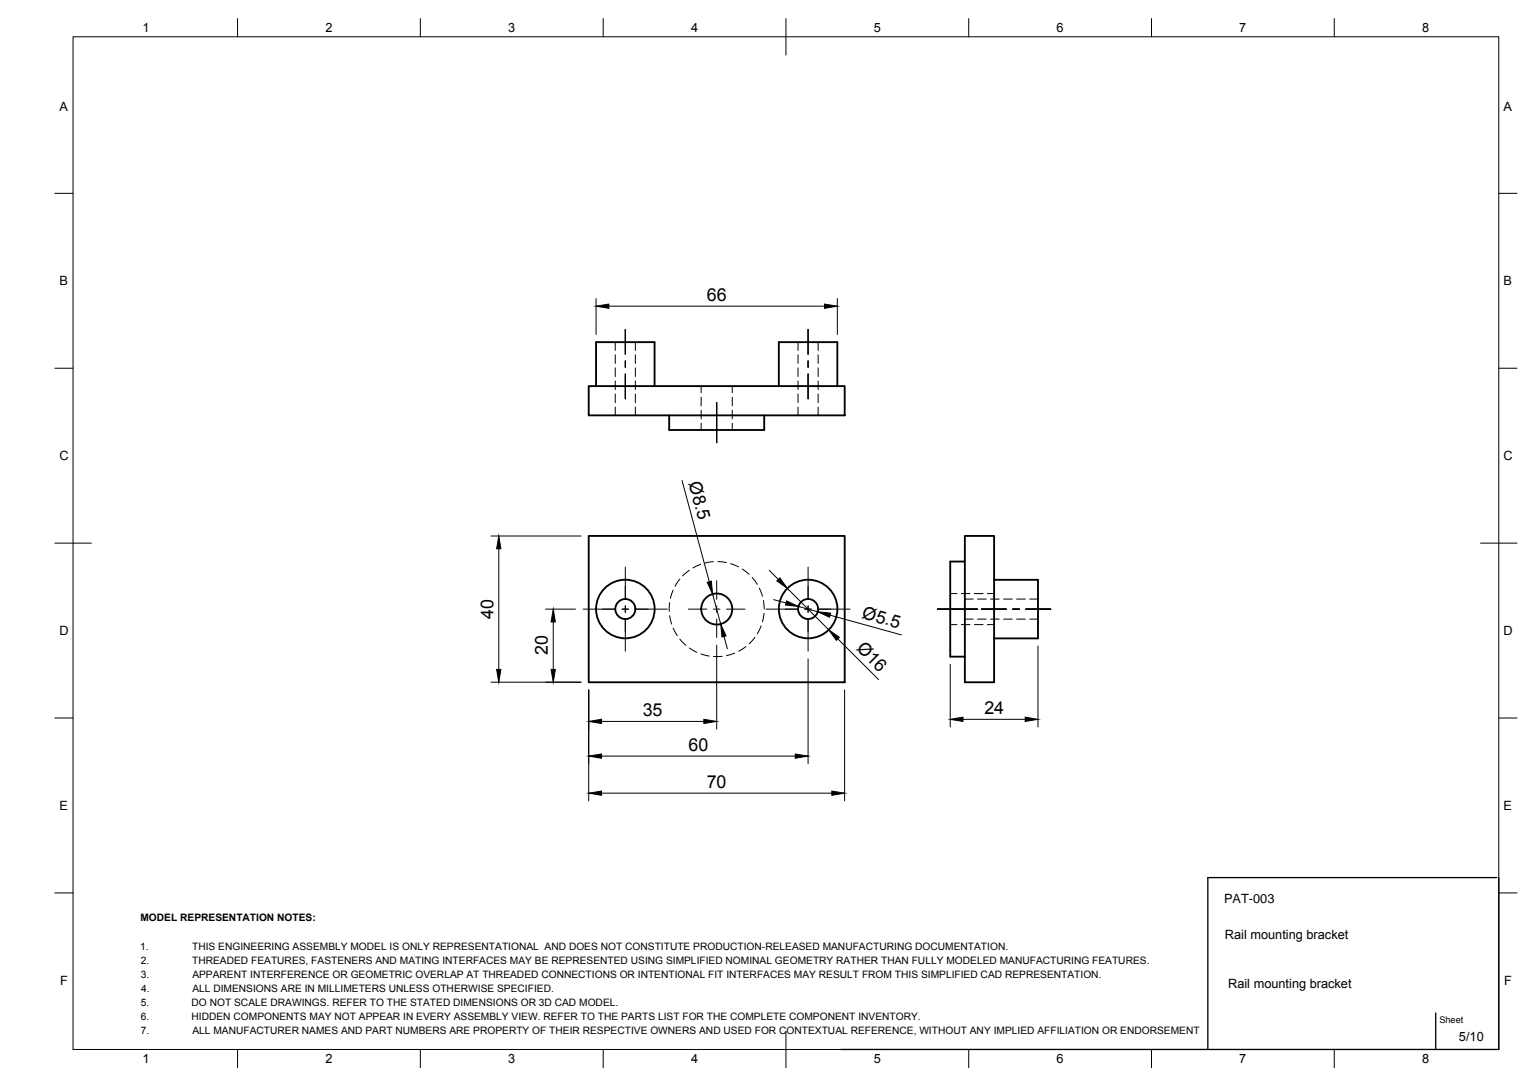
ISO-10303-21;
HEADER;
/* Generated by software containing ST-Developer
 * from STEP Tools, Inc. (www.steptools.com) 
 */

FILE_DESCRIPTION(
/* description */ ('PAT-003'),
/* implementation_level */ '2;1');

FILE_NAME(
/* name */ 'Rail mounting bracket.step',
/* time_stamp */ '2026-10-29T15:45:40-07:00',
/* author */ (''),
/* organization */ (''),
/* preprocessor_version */ 'ST-DEVELOPER v20.2',
/* originating_system */ 'Autodesk Translation Framework v15.17.0.0',
/* authorisation */ '');

FILE_SCHEMA (('AUTOMOTIVE_DESIGN { 1 0 10303 214 3 1 1 }'));
ENDSEC;

DATA;
#10=MECHANICAL_DESIGN_GEOMETRIC_PRESENTATION_REPRESENTATION('',(#147),#5761);
#123=SHAPE_REPRESENTATION_RELATIONSHIP('SRR','None',#5817,#135);
#135=ADVANCED_BREP_SHAPE_REPRESENTATION('',(#159),#5748);
#147=STYLED_ITEM('',(#5928),#159);
#159=MANIFOLD_SOLID_BREP('Body1',#3321);
#169=FACE_BOUND('',#530,.T.);
#170=FACE_BOUND('',#533,.T.);
#171=FACE_BOUND('',#539,.T.);
#172=FACE_BOUND('',#545,.T.);
#173=FACE_BOUND('',#546,.T.);
#174=FACE_BOUND('',#547,.T.);
#175=FACE_BOUND('',#549,.T.);
#176=FACE_BOUND('',#550,.T.);
#177=FACE_BOUND('',#551,.T.);
#206=PLANE('',#3474);
#207=PLANE('',#3479);
#208=PLANE('',#3491);
#209=PLANE('',#3492);
#210=PLANE('',#3493);
#211=PLANE('',#3494);
#212=PLANE('',#3495);
#213=PLANE('',#3496);
#214=PLANE('',#3497);
#341=FACE_OUTER_BOUND('',#528,.T.);
#342=FACE_OUTER_BOUND('',#529,.T.);
#343=FACE_OUTER_BOUND('',#531,.T.);
#344=FACE_OUTER_BOUND('',#532,.T.);
#345=FACE_OUTER_BOUND('',#534,.T.);
#346=FACE_OUTER_BOUND('',#535,.T.);
#347=FACE_OUTER_BOUND('',#536,.T.);
#348=FACE_OUTER_BOUND('',#537,.T.);
#349=FACE_OUTER_BOUND('',#538,.T.);
#350=FACE_OUTER_BOUND('',#540,.T.);
#351=FACE_OUTER_BOUND('',#541,.T.);
#352=FACE_OUTER_BOUND('',#542,.T.);
#353=FACE_OUTER_BOUND('',#543,.T.);
#354=FACE_OUTER_BOUND('',#544,.T.);
#355=FACE_OUTER_BOUND('',#548,.T.);
#528=EDGE_LOOP('',(#2218,#2219,#2220,#2221));
#529=EDGE_LOOP('',(#2222));
#530=EDGE_LOOP('',(#2223));
#531=EDGE_LOOP('',(#2224,#2225,#2226,#2227));
#532=EDGE_LOOP('',(#2228));
#533=EDGE_LOOP('',(#2229));
#534=EDGE_LOOP('',(#2230,#2231,#2232,#2233));
#535=EDGE_LOOP('',(#2234,#2235,#2236,#2237));
#536=EDGE_LOOP('',(#2238,#2239,#2240,#2241));
#537=EDGE_LOOP('',(#2242,#2243,#2244,#2245));
#538=EDGE_LOOP('',(#2246));
#539=EDGE_LOOP('',(#2247));
#540=EDGE_LOOP('',(#2248,#2249,#2250,#2251));
#541=EDGE_LOOP('',(#2252,#2253,#2254,#2255));
#542=EDGE_LOOP('',(#2256,#2257,#2258,#2259));
#543=EDGE_LOOP('',(#2260,#2261,#2262,#2263));
#544=EDGE_LOOP('',(#2264,#2265,#2266,#2267));
#545=EDGE_LOOP('',(#2268));
#546=EDGE_LOOP('',(#2269));
#547=EDGE_LOOP('',(#2270));
#548=EDGE_LOOP('',(#2271,#2272,#2273,#2274));
#549=EDGE_LOOP('',(#2275));
#550=EDGE_LOOP('',(#2276));
#551=EDGE_LOOP('',(#2277));
#752=LINE('',#4754,#1074);
#753=LINE('',#4763,#1075);
#754=LINE('',#4770,#1076);
#755=LINE('',#4774,#1077);
#756=LINE('',#4780,#1078);
#757=LINE('',#4786,#1079);
#758=LINE('',#4792,#1080);
#759=LINE('',#4794,#1081);
#760=LINE('',#4796,#1082);
#761=LINE('',#4797,#1083);
#762=LINE('',#4800,#1084);
#763=LINE('',#4802,#1085);
#764=LINE('',#4803,#1086);
#765=LINE('',#4806,#1087);
#766=LINE('',#4808,#1088);
#767=LINE('',#4809,#1089);
#768=LINE('',#4811,#1090);
#769=LINE('',#4812,#1091);
#1074=VECTOR('',#3797,0.800000000000001);
#1075=VECTOR('',#3808,0.8);
#1076=VECTOR('',#3817,0.275);
#1077=VECTOR('',#3822,0.275);
#1078=VECTOR('',#3829,0.425);
#1079=VECTOR('',#3836,1.3);
#1080=VECTOR('',#3843,1.);
#1081=VECTOR('',#3844,1.);
#1082=VECTOR('',#3845,1.);
#1083=VECTOR('',#3846,1.);
#1084=VECTOR('',#3849,1.);
#1085=VECTOR('',#3850,1.);
#1086=VECTOR('',#3851,1.);
#1087=VECTOR('',#3854,1.);
#1088=VECTOR('',#3855,1.);
#1089=VECTOR('',#3856,1.);
#1090=VECTOR('',#3859,1.);
#1091=VECTOR('',#3860,1.);
#1396=CIRCLE('',#3472,0.800000000000001);
#1397=CIRCLE('',#3473,0.800000000000001);
#1398=CIRCLE('',#3475,0.275);
#1399=CIRCLE('',#3477,0.8);
#1400=CIRCLE('',#3478,0.8);
#1401=CIRCLE('',#3480,0.275);
#1402=CIRCLE('',#3482,0.275);
#1403=CIRCLE('',#3484,0.275);
#1404=CIRCLE('',#3486,0.425);
#1405=CIRCLE('',#3487,0.425);
#1406=CIRCLE('',#3489,1.3);
#1407=CIRCLE('',#3490,1.3);
#1492=VERTEX_POINT('',#4751);
#1493=VERTEX_POINT('',#4753);
#1494=VERTEX_POINT('',#4757);
#1495=VERTEX_POINT('',#4760);
#1496=VERTEX_POINT('',#4762);
#1497=VERTEX_POINT('',#4766);
#1498=VERTEX_POINT('',#4769);
#1499=VERTEX_POINT('',#4773);
#1500=VERTEX_POINT('',#4777);
#1501=VERTEX_POINT('',#4779);
#1502=VERTEX_POINT('',#4783);
#1503=VERTEX_POINT('',#4785);
#1504=VERTEX_POINT('',#4790);
#1505=VERTEX_POINT('',#4791);
#1506=VERTEX_POINT('',#4793);
#1507=VERTEX_POINT('',#4795);
#1508=VERTEX_POINT('',#4799);
#1509=VERTEX_POINT('',#4801);
#1510=VERTEX_POINT('',#4805);
#1511=VERTEX_POINT('',#4807);
#1780=EDGE_CURVE('',#1492,#1492,#1396,.T.);
#1781=EDGE_CURVE('',#1492,#1493,#752,.T.);
#1782=EDGE_CURVE('',#1493,#1493,#1397,.T.);
#1783=EDGE_CURVE('',#1494,#1494,#1398,.T.);
#1784=EDGE_CURVE('',#1495,#1495,#1399,.T.);
#1785=EDGE_CURVE('',#1495,#1496,#753,.T.);
#1786=EDGE_CURVE('',#1496,#1496,#1400,.T.);
#1787=EDGE_CURVE('',#1497,#1497,#1401,.T.);
#1788=EDGE_CURVE('',#1497,#1498,#754,.T.);
#1789=EDGE_CURVE('',#1498,#1498,#1402,.T.);
#1790=EDGE_CURVE('',#1494,#1499,#755,.T.);
#1791=EDGE_CURVE('',#1499,#1499,#1403,.T.);
#1792=EDGE_CURVE('',#1500,#1500,#1404,.T.);
#1793=EDGE_CURVE('',#1500,#1501,#756,.T.);
#1794=EDGE_CURVE('',#1501,#1501,#1405,.T.);
#1795=EDGE_CURVE('',#1502,#1502,#1406,.T.);
#1796=EDGE_CURVE('',#1502,#1503,#757,.T.);
#1797=EDGE_CURVE('',#1503,#1503,#1407,.T.);
#1798=EDGE_CURVE('',#1504,#1505,#758,.T.);
#1799=EDGE_CURVE('',#1505,#1506,#759,.T.);
#1800=EDGE_CURVE('',#1507,#1506,#760,.T.);
#1801=EDGE_CURVE('',#1504,#1507,#761,.T.);
#1802=EDGE_CURVE('',#1508,#1504,#762,.T.);
#1803=EDGE_CURVE('',#1509,#1507,#763,.T.);
#1804=EDGE_CURVE('',#1508,#1509,#764,.T.);
#1805=EDGE_CURVE('',#1510,#1508,#765,.T.);
#1806=EDGE_CURVE('',#1511,#1509,#766,.T.);
#1807=EDGE_CURVE('',#1510,#1511,#767,.T.);
#1808=EDGE_CURVE('',#1505,#1510,#768,.T.);
#1809=EDGE_CURVE('',#1506,#1511,#769,.T.);
#2218=ORIENTED_EDGE('',*,*,#1780,.F.);
#2219=ORIENTED_EDGE('',*,*,#1781,.T.);
#2220=ORIENTED_EDGE('',*,*,#1782,.T.);
#2221=ORIENTED_EDGE('',*,*,#1781,.F.);
#2222=ORIENTED_EDGE('',*,*,#1782,.F.);
#2223=ORIENTED_EDGE('',*,*,#1783,.F.);
#2224=ORIENTED_EDGE('',*,*,#1784,.F.);
#2225=ORIENTED_EDGE('',*,*,#1785,.T.);
#2226=ORIENTED_EDGE('',*,*,#1786,.T.);
#2227=ORIENTED_EDGE('',*,*,#1785,.F.);
#2228=ORIENTED_EDGE('',*,*,#1786,.F.);
#2229=ORIENTED_EDGE('',*,*,#1787,.F.);
#2230=ORIENTED_EDGE('',*,*,#1787,.T.);
#2231=ORIENTED_EDGE('',*,*,#1788,.T.);
#2232=ORIENTED_EDGE('',*,*,#1789,.F.);
#2233=ORIENTED_EDGE('',*,*,#1788,.F.);
#2234=ORIENTED_EDGE('',*,*,#1783,.T.);
#2235=ORIENTED_EDGE('',*,*,#1790,.T.);
#2236=ORIENTED_EDGE('',*,*,#1791,.F.);
#2237=ORIENTED_EDGE('',*,*,#1790,.F.);
#2238=ORIENTED_EDGE('',*,*,#1792,.F.);
#2239=ORIENTED_EDGE('',*,*,#1793,.T.);
#2240=ORIENTED_EDGE('',*,*,#1794,.F.);
#2241=ORIENTED_EDGE('',*,*,#1793,.F.);
#2242=ORIENTED_EDGE('',*,*,#1795,.F.);
#2243=ORIENTED_EDGE('',*,*,#1796,.T.);
#2244=ORIENTED_EDGE('',*,*,#1797,.F.);
#2245=ORIENTED_EDGE('',*,*,#1796,.F.);
#2246=ORIENTED_EDGE('',*,*,#1795,.T.);
#2247=ORIENTED_EDGE('',*,*,#1794,.T.);
#2248=ORIENTED_EDGE('',*,*,#1798,.T.);
#2249=ORIENTED_EDGE('',*,*,#1799,.T.);
#2250=ORIENTED_EDGE('',*,*,#1800,.F.);
#2251=ORIENTED_EDGE('',*,*,#1801,.F.);
#2252=ORIENTED_EDGE('',*,*,#1802,.T.);
#2253=ORIENTED_EDGE('',*,*,#1801,.T.);
#2254=ORIENTED_EDGE('',*,*,#1803,.F.);
#2255=ORIENTED_EDGE('',*,*,#1804,.F.);
#2256=ORIENTED_EDGE('',*,*,#1805,.T.);
#2257=ORIENTED_EDGE('',*,*,#1804,.T.);
#2258=ORIENTED_EDGE('',*,*,#1806,.F.);
#2259=ORIENTED_EDGE('',*,*,#1807,.F.);
#2260=ORIENTED_EDGE('',*,*,#1808,.T.);
#2261=ORIENTED_EDGE('',*,*,#1807,.T.);
#2262=ORIENTED_EDGE('',*,*,#1809,.F.);
#2263=ORIENTED_EDGE('',*,*,#1799,.F.);
#2264=ORIENTED_EDGE('',*,*,#1809,.T.);
#2265=ORIENTED_EDGE('',*,*,#1806,.T.);
#2266=ORIENTED_EDGE('',*,*,#1803,.T.);
#2267=ORIENTED_EDGE('',*,*,#1800,.T.);
#2268=ORIENTED_EDGE('',*,*,#1789,.T.);
#2269=ORIENTED_EDGE('',*,*,#1791,.T.);
#2270=ORIENTED_EDGE('',*,*,#1797,.T.);
#2271=ORIENTED_EDGE('',*,*,#1808,.F.);
#2272=ORIENTED_EDGE('',*,*,#1798,.F.);
#2273=ORIENTED_EDGE('',*,*,#1802,.F.);
#2274=ORIENTED_EDGE('',*,*,#1805,.F.);
#2275=ORIENTED_EDGE('',*,*,#1780,.T.);
#2276=ORIENTED_EDGE('',*,*,#1784,.T.);
#2277=ORIENTED_EDGE('',*,*,#1792,.T.);
#3094=CYLINDRICAL_SURFACE('',#3471,0.800000000000001);
#3095=CYLINDRICAL_SURFACE('',#3476,0.8);
#3096=CYLINDRICAL_SURFACE('',#3481,0.275);
#3097=CYLINDRICAL_SURFACE('',#3483,0.275);
#3098=CYLINDRICAL_SURFACE('',#3485,0.425);
#3099=CYLINDRICAL_SURFACE('',#3488,1.3);
#3134=ADVANCED_FACE('',(#341),#3094,.T.);
#3135=ADVANCED_FACE('',(#342,#169),#206,.F.);
#3136=ADVANCED_FACE('',(#343),#3095,.T.);
#3137=ADVANCED_FACE('',(#344,#170),#207,.F.);
#3138=ADVANCED_FACE('',(#345),#3096,.F.);
#3139=ADVANCED_FACE('',(#346),#3097,.F.);
#3140=ADVANCED_FACE('',(#347),#3098,.F.);
#3141=ADVANCED_FACE('',(#348),#3099,.T.);
#3142=ADVANCED_FACE('',(#349,#171),#208,.T.);
#3143=ADVANCED_FACE('',(#350),#209,.T.);
#3144=ADVANCED_FACE('',(#351),#210,.T.);
#3145=ADVANCED_FACE('',(#352),#211,.T.);
#3146=ADVANCED_FACE('',(#353),#212,.T.);
#3147=ADVANCED_FACE('',(#354,#172,#173,#174),#213,.T.);
#3148=ADVANCED_FACE('',(#355,#175,#176,#177),#214,.F.);
#3321=CLOSED_SHELL('',(#3134,#3135,#3136,#3137,#3138,#3139,#3140,#3141,
#3142,#3143,#3144,#3145,#3146,#3147,#3148));
#3470=AXIS2_PLACEMENT_3D('',#4749,#3791,#3792);
#3471=AXIS2_PLACEMENT_3D('',#4750,#3793,#3794);
#3472=AXIS2_PLACEMENT_3D('',#4752,#3795,#3796);
#3473=AXIS2_PLACEMENT_3D('',#4755,#3798,#3799);
#3474=AXIS2_PLACEMENT_3D('',#4756,#3800,#3801);
#3475=AXIS2_PLACEMENT_3D('',#4758,#3802,#3803);
#3476=AXIS2_PLACEMENT_3D('',#4759,#3804,#3805);
#3477=AXIS2_PLACEMENT_3D('',#4761,#3806,#3807);
#3478=AXIS2_PLACEMENT_3D('',#4764,#3809,#3810);
#3479=AXIS2_PLACEMENT_3D('',#4765,#3811,#3812);
#3480=AXIS2_PLACEMENT_3D('',#4767,#3813,#3814);
#3481=AXIS2_PLACEMENT_3D('',#4768,#3815,#3816);
#3482=AXIS2_PLACEMENT_3D('',#4771,#3818,#3819);
#3483=AXIS2_PLACEMENT_3D('',#4772,#3820,#3821);
#3484=AXIS2_PLACEMENT_3D('',#4775,#3823,#3824);
#3485=AXIS2_PLACEMENT_3D('',#4776,#3825,#3826);
#3486=AXIS2_PLACEMENT_3D('',#4778,#3827,#3828);
#3487=AXIS2_PLACEMENT_3D('',#4781,#3830,#3831);
#3488=AXIS2_PLACEMENT_3D('',#4782,#3832,#3833);
#3489=AXIS2_PLACEMENT_3D('',#4784,#3834,#3835);
#3490=AXIS2_PLACEMENT_3D('',#4787,#3837,#3838);
#3491=AXIS2_PLACEMENT_3D('',#4788,#3839,#3840);
#3492=AXIS2_PLACEMENT_3D('',#4789,#3841,#3842);
#3493=AXIS2_PLACEMENT_3D('',#4798,#3847,#3848);
#3494=AXIS2_PLACEMENT_3D('',#4804,#3852,#3853);
#3495=AXIS2_PLACEMENT_3D('',#4810,#3857,#3858);
#3496=AXIS2_PLACEMENT_3D('',#4813,#3861,#3862);
#3497=AXIS2_PLACEMENT_3D('',#4814,#3863,#3864);
#3791=DIRECTION('axis',(0.,0.,1.));
#3792=DIRECTION('refdir',(1.,0.,0.));
#3793=DIRECTION('center_axis',(0.,0.,1.));
#3794=DIRECTION('ref_axis',(1.,0.,0.));
#3795=DIRECTION('center_axis',(0.,0.,1.));
#3796=DIRECTION('ref_axis',(1.,0.,0.));
#3797=DIRECTION('',(0.,0.,-1.));
#3798=DIRECTION('center_axis',(0.,0.,1.));
#3799=DIRECTION('ref_axis',(1.,0.,0.));
#3800=DIRECTION('center_axis',(0.,0.,1.));
#3801=DIRECTION('ref_axis',(1.,0.,0.));
#3802=DIRECTION('center_axis',(0.,0.,-1.));
#3803=DIRECTION('ref_axis',(1.,0.,0.));
#3804=DIRECTION('center_axis',(0.,0.,1.));
#3805=DIRECTION('ref_axis',(1.,0.,0.));
#3806=DIRECTION('center_axis',(0.,0.,1.));
#3807=DIRECTION('ref_axis',(1.,0.,0.));
#3808=DIRECTION('',(0.,0.,-1.));
#3809=DIRECTION('center_axis',(0.,0.,1.));
#3810=DIRECTION('ref_axis',(1.,0.,0.));
#3811=DIRECTION('center_axis',(0.,0.,1.));
#3812=DIRECTION('ref_axis',(1.,0.,0.));
#3813=DIRECTION('center_axis',(0.,0.,-1.));
#3814=DIRECTION('ref_axis',(1.,0.,0.));
#3815=DIRECTION('center_axis',(0.,0.,1.));
#3816=DIRECTION('ref_axis',(1.,0.,0.));
#3817=DIRECTION('',(0.,0.,1.));
#3818=DIRECTION('center_axis',(0.,0.,-1.));
#3819=DIRECTION('ref_axis',(1.,0.,0.));
#3820=DIRECTION('center_axis',(0.,0.,1.));
#3821=DIRECTION('ref_axis',(1.,0.,0.));
#3822=DIRECTION('',(0.,0.,1.));
#3823=DIRECTION('center_axis',(0.,0.,-1.));
#3824=DIRECTION('ref_axis',(1.,0.,0.));
#3825=DIRECTION('center_axis',(0.,0.,1.));
#3826=DIRECTION('ref_axis',(1.,0.,0.));
#3827=DIRECTION('center_axis',(0.,0.,1.));
#3828=DIRECTION('ref_axis',(1.,0.,0.));
#3829=DIRECTION('',(0.,0.,1.));
#3830=DIRECTION('center_axis',(0.,0.,-1.));
#3831=DIRECTION('ref_axis',(1.,0.,0.));
#3832=DIRECTION('center_axis',(0.,0.,1.));
#3833=DIRECTION('ref_axis',(1.,0.,0.));
#3834=DIRECTION('center_axis',(0.,0.,1.));
#3835=DIRECTION('ref_axis',(1.,0.,0.));
#3836=DIRECTION('',(0.,0.,-1.));
#3837=DIRECTION('center_axis',(0.,0.,-1.));
#3838=DIRECTION('ref_axis',(1.,0.,0.));
#3839=DIRECTION('center_axis',(0.,0.,1.));
#3840=DIRECTION('ref_axis',(1.,0.,0.));
#3841=DIRECTION('center_axis',(0.,1.,0.));
#3842=DIRECTION('ref_axis',(-1.,0.,0.));
#3843=DIRECTION('',(-1.,0.,0.));
#3844=DIRECTION('',(0.,0.,1.));
#3845=DIRECTION('',(-1.,0.,0.));
#3846=DIRECTION('',(0.,0.,1.));
#3847=DIRECTION('center_axis',(1.,0.,0.));
#3848=DIRECTION('ref_axis',(0.,1.,0.));
#3849=DIRECTION('',(0.,1.,0.));
#3850=DIRECTION('',(0.,1.,0.));
#3851=DIRECTION('',(0.,0.,1.));
#3852=DIRECTION('center_axis',(0.,-1.,0.));
#3853=DIRECTION('ref_axis',(1.,0.,0.));
#3854=DIRECTION('',(1.,0.,0.));
#3855=DIRECTION('',(1.,0.,0.));
#3856=DIRECTION('',(0.,0.,1.));
#3857=DIRECTION('center_axis',(-1.,0.,0.));
#3858=DIRECTION('ref_axis',(0.,-1.,0.));
#3859=DIRECTION('',(0.,-1.,0.));
#3860=DIRECTION('',(0.,-1.,0.));
#3861=DIRECTION('center_axis',(0.,0.,1.));
#3862=DIRECTION('ref_axis',(1.,0.,0.));
#3863=DIRECTION('center_axis',(0.,0.,1.));
#3864=DIRECTION('ref_axis',(1.,0.,0.));
#4749=CARTESIAN_POINT('',(0.,0.,0.));
#4750=CARTESIAN_POINT('Origin',(7.5,0.,2.));
#4751=CARTESIAN_POINT('',(6.7,-9.79717439317883E-17,3.2));
#4752=CARTESIAN_POINT('Origin',(7.5,0.,3.2));
#4753=CARTESIAN_POINT('',(6.7,-9.79717439317883E-17,2.));
#4754=CARTESIAN_POINT('',(6.7,-9.79717439317883E-17,2.));
#4755=CARTESIAN_POINT('Origin',(7.5,0.,2.));
#4756=CARTESIAN_POINT('Origin',(7.5,0.,2.));
#4757=CARTESIAN_POINT('',(7.225,-3.36777869765523E-17,2.));
#4758=CARTESIAN_POINT('Origin',(7.5,0.,2.));
#4759=CARTESIAN_POINT('Origin',(2.5,0.,2.));
#4760=CARTESIAN_POINT('',(1.7,-9.79717439317882E-17,3.2));
#4761=CARTESIAN_POINT('Origin',(2.5,0.,3.2));
#4762=CARTESIAN_POINT('',(1.7,-9.79717439317882E-17,2.));
#4763=CARTESIAN_POINT('',(1.7,-9.79717439317882E-17,2.));
#4764=CARTESIAN_POINT('Origin',(2.5,0.,2.));
#4765=CARTESIAN_POINT('Origin',(2.5,0.,2.));
#4766=CARTESIAN_POINT('',(2.225,-3.36777869765522E-17,2.));
#4767=CARTESIAN_POINT('Origin',(2.5,0.,2.));
#4768=CARTESIAN_POINT('Origin',(2.5,0.,3.1));
#4769=CARTESIAN_POINT('',(2.225,3.36777869765522E-17,4.));
#4770=CARTESIAN_POINT('',(2.225,-3.36777869765522E-17,3.1));
#4771=CARTESIAN_POINT('Origin',(2.5,0.,4.));
#4772=CARTESIAN_POINT('Origin',(7.5,0.,3.1));
#4773=CARTESIAN_POINT('',(7.225,3.36777869765523E-17,4.));
#4774=CARTESIAN_POINT('',(7.225,-3.36777869765523E-17,3.1));
#4775=CARTESIAN_POINT('Origin',(7.5,0.,4.));
#4776=CARTESIAN_POINT('Origin',(5.,0.,3.1));
#4777=CARTESIAN_POINT('',(4.575,-5.20474889637625E-17,3.2));
#4778=CARTESIAN_POINT('Origin',(5.,0.,3.2));
#4779=CARTESIAN_POINT('',(4.575,5.20474889637625E-17,4.4));
#4780=CARTESIAN_POINT('',(4.575,-5.20474889637625E-17,3.1));
#4781=CARTESIAN_POINT('Origin',(5.,0.,4.4));
#4782=CARTESIAN_POINT('Origin',(5.,0.,4.));
#4783=CARTESIAN_POINT('',(3.7,-1.59204083889156E-16,4.4));
#4784=CARTESIAN_POINT('Origin',(5.,0.,4.4));
#4785=CARTESIAN_POINT('',(3.7,-1.59204083889156E-16,4.));
#4786=CARTESIAN_POINT('',(3.7,-1.59204083889156E-16,4.));
#4787=CARTESIAN_POINT('Origin',(5.,0.,4.));
#4788=CARTESIAN_POINT('Origin',(5.,0.,4.4));
#4789=CARTESIAN_POINT('Origin',(8.5,2.,3.2));
#4790=CARTESIAN_POINT('',(8.5,2.,3.2));
#4791=CARTESIAN_POINT('',(1.5,2.,3.2));
#4792=CARTESIAN_POINT('',(8.5,2.,3.2));
#4793=CARTESIAN_POINT('',(1.5,2.,4.));
#4794=CARTESIAN_POINT('',(1.5,2.,3.2));
#4795=CARTESIAN_POINT('',(8.5,2.,4.));
#4796=CARTESIAN_POINT('',(8.5,2.,4.));
#4797=CARTESIAN_POINT('',(8.5,2.,3.2));
#4798=CARTESIAN_POINT('Origin',(8.5,-2.,3.2));
#4799=CARTESIAN_POINT('',(8.5,-2.,3.2));
#4800=CARTESIAN_POINT('',(8.5,-2.,3.2));
#4801=CARTESIAN_POINT('',(8.5,-2.,4.));
#4802=CARTESIAN_POINT('',(8.5,-2.,4.));
#4803=CARTESIAN_POINT('',(8.5,-2.,3.2));
#4804=CARTESIAN_POINT('Origin',(1.5,-2.,3.2));
#4805=CARTESIAN_POINT('',(1.5,-2.,3.2));
#4806=CARTESIAN_POINT('',(1.5,-2.,3.2));
#4807=CARTESIAN_POINT('',(1.5,-2.,4.));
#4808=CARTESIAN_POINT('',(1.5,-2.,4.));
#4809=CARTESIAN_POINT('',(1.5,-2.,3.2));
#4810=CARTESIAN_POINT('Origin',(1.5,2.,3.2));
#4811=CARTESIAN_POINT('',(1.5,2.,3.2));
#4812=CARTESIAN_POINT('',(1.5,2.,4.));
#4813=CARTESIAN_POINT('Origin',(5.,0.,4.));
#4814=CARTESIAN_POINT('Origin',(5.,0.,3.2));
#5732=UNCERTAINTY_MEASURE_WITH_UNIT(LENGTH_MEASURE(0.001),#5762,
'DISTANCE_ACCURACY_VALUE',
'Maximum model space distance between geometric entities at asserted c
onnectivities');
#5745=UNCERTAINTY_MEASURE_WITH_UNIT(LENGTH_MEASURE(0.001),#5762,
'DISTANCE_ACCURACY_VALUE',
'Maximum model space distance between geometric entities at asserted c
onnectivities');
#5748=(
GEOMETRIC_REPRESENTATION_CONTEXT(3)
GLOBAL_UNCERTAINTY_ASSIGNED_CONTEXT((#5732))
GLOBAL_UNIT_ASSIGNED_CONTEXT((#5762,#5764,#5765))
REPRESENTATION_CONTEXT('','3D')
);
#5761=(
GEOMETRIC_REPRESENTATION_CONTEXT(3)
GLOBAL_UNCERTAINTY_ASSIGNED_CONTEXT((#5745))
GLOBAL_UNIT_ASSIGNED_CONTEXT((#5762,#5764,#5765))
REPRESENTATION_CONTEXT('','3D')
);
#5762=(
LENGTH_UNIT()
NAMED_UNIT(*)
SI_UNIT(.CENTI.,.METRE.)
);
#5764=(
NAMED_UNIT(*)
PLANE_ANGLE_UNIT()
SI_UNIT($,.RADIAN.)
);
#5765=(
NAMED_UNIT(*)
SI_UNIT($,.STERADIAN.)
SOLID_ANGLE_UNIT()
);
#5768=SHAPE_DEFINITION_REPRESENTATION(#5783,#5817);
#5783=PRODUCT_DEFINITION_SHAPE('',$,#5833);
#5817=SHAPE_REPRESENTATION('',(#3470),#5748);
#5830=PRODUCT_DEFINITION_CONTEXT('part definition',#5877,'design');
#5833=PRODUCT_DEFINITION('Rail mounting bracket',
'Rail mounting bracket',#5848,#5830);
#5848=PRODUCT_DEFINITION_FORMATION('',$,#5881);
#5877=APPLICATION_CONTEXT(
'Core Data for Automotive Mechanical Design Process');
#5878=PRODUCT_CONTEXT('part definition',#5877,'mechanical');
#5881=PRODUCT('Rail mounting bracket','Rail mounting bracket',
'Rail mounting bracket',(#5878));
#5922=COLOUR_RGB('Dark Blue',0.08,0.2,0.34);
#5923=FILL_AREA_STYLE_COLOUR('',#5922);
#5924=FILL_AREA_STYLE('',(#5923));
#5925=SURFACE_STYLE_FILL_AREA(#5924);
#5926=SURFACE_SIDE_STYLE('',(#5925));
#5927=SURFACE_STYLE_USAGE(.BOTH.,#5926);
#5928=PRESENTATION_STYLE_ASSIGNMENT((#5927));
ENDSEC;
END-ISO-10303-21;
